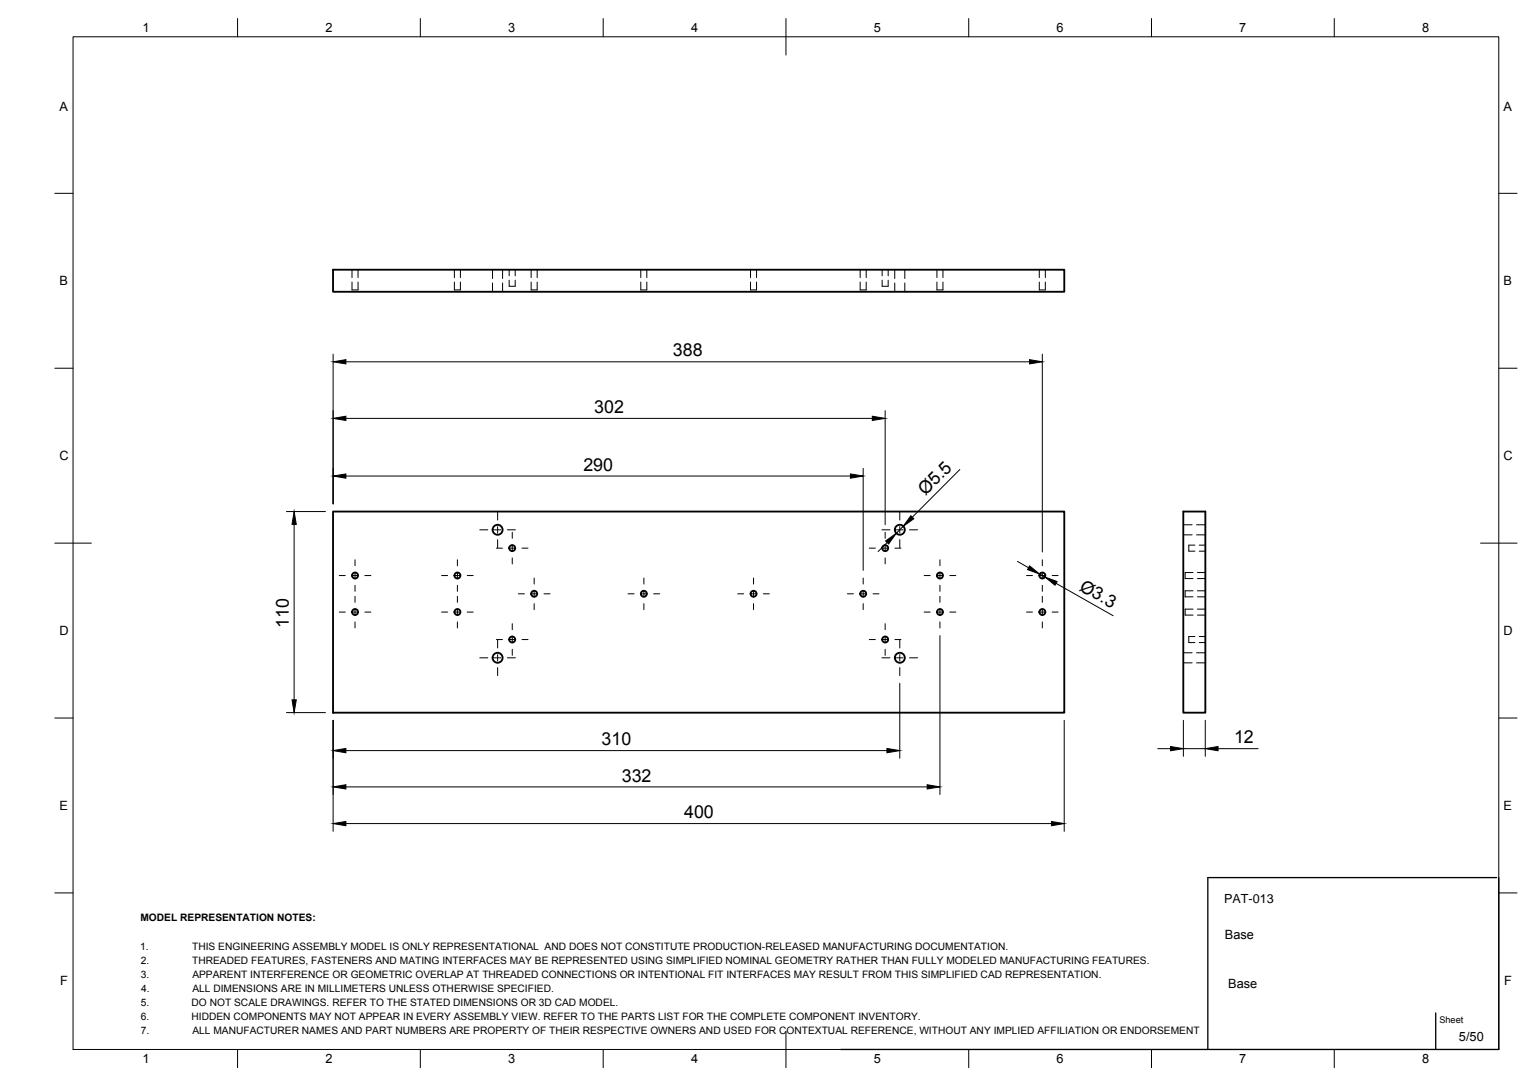
ISO-10303-21;
HEADER;
/* Generated by software containing ST-Developer
 * from STEP Tools, Inc. (www.steptools.com) 
 */

FILE_DESCRIPTION(
/* description */ ('Belt-driven linear axis on 2020 extrusion'),
/* implementation_level */ '2;1');

FILE_NAME(
/* name */ 'Base.step',
/* time_stamp */ '2026-10-28T03:26:09-07:00',
/* author */ (''),
/* organization */ (''),
/* preprocessor_version */ 'ST-DEVELOPER v20.2',
/* originating_system */ 'Autodesk Translation Framework v15.17.0.0',
/* authorisation */ '');

FILE_SCHEMA (('AUTOMOTIVE_DESIGN { 1 0 10303 214 3 1 1 }'));
ENDSEC;

DATA;
#10=MECHANICAL_DESIGN_GEOMETRIC_PRESENTATION_REPRESENTATION('',(#610),#20096);
#518=SHAPE_REPRESENTATION_RELATIONSHIP('SRR','None',#20314,#564);
#564=ADVANCED_BREP_SHAPE_REPRESENTATION('',(#666),#20045);
#610=STYLED_ITEM('',(#20629),#666);
#666=MANIFOLD_SOLID_BREP('Body1',#10923);
#718=FACE_BOUND('',#1913,.T.);
#719=FACE_BOUND('',#1914,.T.);
#720=FACE_BOUND('',#1915,.T.);
#721=FACE_BOUND('',#1916,.T.);
#722=FACE_BOUND('',#1917,.T.);
#723=FACE_BOUND('',#1918,.T.);
#724=FACE_BOUND('',#1919,.T.);
#725=FACE_BOUND('',#1920,.T.);
#726=FACE_BOUND('',#1921,.T.);
#727=FACE_BOUND('',#1922,.T.);
#728=FACE_BOUND('',#1923,.T.);
#729=FACE_BOUND('',#1924,.T.);
#730=FACE_BOUND('',#1925,.T.);
#731=FACE_BOUND('',#1926,.T.);
#732=FACE_BOUND('',#1927,.T.);
#733=FACE_BOUND('',#1928,.T.);
#734=FACE_BOUND('',#1929,.T.);
#735=FACE_BOUND('',#1930,.T.);
#736=FACE_BOUND('',#1931,.T.);
#737=FACE_BOUND('',#1932,.T.);
#738=FACE_BOUND('',#1934,.T.);
#739=FACE_BOUND('',#1935,.T.);
#740=FACE_BOUND('',#1936,.T.);
#741=FACE_BOUND('',#1937,.T.);
#889=PLANE('',#11496);
#890=PLANE('',#11500);
#891=PLANE('',#11504);
#892=PLANE('',#11508);
#893=PLANE('',#11512);
#894=PLANE('',#11516);
#895=PLANE('',#11520);
#896=PLANE('',#11524);
#897=PLANE('',#11540);
#898=PLANE('',#11544);
#899=PLANE('',#11548);
#900=PLANE('',#11552);
#901=PLANE('',#11556);
#902=PLANE('',#11560);
#903=PLANE('',#11564);
#904=PLANE('',#11568);
#905=PLANE('',#11569);
#906=PLANE('',#11570);
#907=PLANE('',#11571);
#908=PLANE('',#11572);
#909=PLANE('',#11573);
#910=PLANE('',#11574);
#1250=FACE_OUTER_BOUND('',#1872,.T.);
#1251=FACE_OUTER_BOUND('',#1873,.T.);
#1252=FACE_OUTER_BOUND('',#1874,.T.);
#1253=FACE_OUTER_BOUND('',#1875,.T.);
#1254=FACE_OUTER_BOUND('',#1876,.T.);
#1255=FACE_OUTER_BOUND('',#1877,.T.);
#1256=FACE_OUTER_BOUND('',#1878,.T.);
#1257=FACE_OUTER_BOUND('',#1879,.T.);
#1258=FACE_OUTER_BOUND('',#1880,.T.);
#1259=FACE_OUTER_BOUND('',#1881,.T.);
#1260=FACE_OUTER_BOUND('',#1882,.T.);
#1261=FACE_OUTER_BOUND('',#1883,.T.);
#1262=FACE_OUTER_BOUND('',#1884,.T.);
#1263=FACE_OUTER_BOUND('',#1885,.T.);
#1264=FACE_OUTER_BOUND('',#1886,.T.);
#1265=FACE_OUTER_BOUND('',#1887,.T.);
#1266=FACE_OUTER_BOUND('',#1888,.T.);
#1267=FACE_OUTER_BOUND('',#1889,.T.);
#1268=FACE_OUTER_BOUND('',#1890,.T.);
#1269=FACE_OUTER_BOUND('',#1891,.T.);
#1270=FACE_OUTER_BOUND('',#1892,.T.);
#1271=FACE_OUTER_BOUND('',#1893,.T.);
#1272=FACE_OUTER_BOUND('',#1894,.T.);
#1273=FACE_OUTER_BOUND('',#1895,.T.);
#1274=FACE_OUTER_BOUND('',#1896,.T.);
#1275=FACE_OUTER_BOUND('',#1897,.T.);
#1276=FACE_OUTER_BOUND('',#1898,.T.);
#1277=FACE_OUTER_BOUND('',#1899,.T.);
#1278=FACE_OUTER_BOUND('',#1900,.T.);
#1279=FACE_OUTER_BOUND('',#1901,.T.);
#1280=FACE_OUTER_BOUND('',#1902,.T.);
#1281=FACE_OUTER_BOUND('',#1903,.T.);
#1282=FACE_OUTER_BOUND('',#1904,.T.);
#1283=FACE_OUTER_BOUND('',#1905,.T.);
#1284=FACE_OUTER_BOUND('',#1906,.T.);
#1285=FACE_OUTER_BOUND('',#1907,.T.);
#1286=FACE_OUTER_BOUND('',#1908,.T.);
#1287=FACE_OUTER_BOUND('',#1909,.T.);
#1288=FACE_OUTER_BOUND('',#1910,.T.);
#1289=FACE_OUTER_BOUND('',#1911,.T.);
#1290=FACE_OUTER_BOUND('',#1912,.T.);
#1291=FACE_OUTER_BOUND('',#1933,.T.);
#1872=EDGE_LOOP('',(#7253,#7254,#7255,#7256));
#1873=EDGE_LOOP('',(#7257));
#1874=EDGE_LOOP('',(#7258,#7259,#7260,#7261));
#1875=EDGE_LOOP('',(#7262));
#1876=EDGE_LOOP('',(#7263,#7264,#7265,#7266));
#1877=EDGE_LOOP('',(#7267));
#1878=EDGE_LOOP('',(#7268,#7269,#7270,#7271));
#1879=EDGE_LOOP('',(#7272));
#1880=EDGE_LOOP('',(#7273,#7274,#7275,#7276));
#1881=EDGE_LOOP('',(#7277));
#1882=EDGE_LOOP('',(#7278,#7279,#7280,#7281));
#1883=EDGE_LOOP('',(#7282));
#1884=EDGE_LOOP('',(#7283,#7284,#7285,#7286));
#1885=EDGE_LOOP('',(#7287));
#1886=EDGE_LOOP('',(#7288,#7289,#7290,#7291));
#1887=EDGE_LOOP('',(#7292));
#1888=EDGE_LOOP('',(#7293,#7294,#7295,#7296));
#1889=EDGE_LOOP('',(#7297,#7298,#7299,#7300));
#1890=EDGE_LOOP('',(#7301,#7302,#7303,#7304));
#1891=EDGE_LOOP('',(#7305,#7306,#7307,#7308));
#1892=EDGE_LOOP('',(#7309,#7310,#7311,#7312));
#1893=EDGE_LOOP('',(#7313));
#1894=EDGE_LOOP('',(#7314,#7315,#7316,#7317));
#1895=EDGE_LOOP('',(#7318));
#1896=EDGE_LOOP('',(#7319,#7320,#7321,#7322));
#1897=EDGE_LOOP('',(#7323));
#1898=EDGE_LOOP('',(#7324,#7325,#7326,#7327));
#1899=EDGE_LOOP('',(#7328));
#1900=EDGE_LOOP('',(#7329,#7330,#7331,#7332));
#1901=EDGE_LOOP('',(#7333));
#1902=EDGE_LOOP('',(#7334,#7335,#7336,#7337));
#1903=EDGE_LOOP('',(#7338));
#1904=EDGE_LOOP('',(#7339,#7340,#7341,#7342));
#1905=EDGE_LOOP('',(#7343));
#1906=EDGE_LOOP('',(#7344,#7345,#7346,#7347));
#1907=EDGE_LOOP('',(#7348));
#1908=EDGE_LOOP('',(#7349,#7350,#7351,#7352));
#1909=EDGE_LOOP('',(#7353,#7354,#7355,#7356));
#1910=EDGE_LOOP('',(#7357,#7358,#7359,#7360));
#1911=EDGE_LOOP('',(#7361,#7362,#7363,#7364));
#1912=EDGE_LOOP('',(#7365,#7366,#7367,#7368));
#1913=EDGE_LOOP('',(#7369));
#1914=EDGE_LOOP('',(#7370));
#1915=EDGE_LOOP('',(#7371));
#1916=EDGE_LOOP('',(#7372));
#1917=EDGE_LOOP('',(#7373));
#1918=EDGE_LOOP('',(#7374));
#1919=EDGE_LOOP('',(#7375));
#1920=EDGE_LOOP('',(#7376));
#1921=EDGE_LOOP('',(#7377));
#1922=EDGE_LOOP('',(#7378));
#1923=EDGE_LOOP('',(#7379));
#1924=EDGE_LOOP('',(#7380));
#1925=EDGE_LOOP('',(#7381));
#1926=EDGE_LOOP('',(#7382));
#1927=EDGE_LOOP('',(#7383));
#1928=EDGE_LOOP('',(#7384));
#1929=EDGE_LOOP('',(#7385));
#1930=EDGE_LOOP('',(#7386));
#1931=EDGE_LOOP('',(#7387));
#1932=EDGE_LOOP('',(#7388));
#1933=EDGE_LOOP('',(#7389,#7390,#7391,#7392));
#1934=EDGE_LOOP('',(#7393));
#1935=EDGE_LOOP('',(#7394));
#1936=EDGE_LOOP('',(#7395));
#1937=EDGE_LOOP('',(#7396));
#2665=LINE('',#16239,#3522);
#2666=LINE('',#16246,#3523);
#2667=LINE('',#16253,#3524);
#2668=LINE('',#16260,#3525);
#2669=LINE('',#16267,#3526);
#2670=LINE('',#16274,#3527);
#2671=LINE('',#16281,#3528);
#2672=LINE('',#16288,#3529);
#2673=LINE('',#16295,#3530);
#2674=LINE('',#16301,#3531);
#2675=LINE('',#16307,#3532);
#2676=LINE('',#16313,#3533);
#2677=LINE('',#16319,#3534);
#2678=LINE('',#16326,#3535);
#2679=LINE('',#16333,#3536);
#2680=LINE('',#16340,#3537);
#2681=LINE('',#16347,#3538);
#2682=LINE('',#16354,#3539);
#2683=LINE('',#16361,#3540);
#2684=LINE('',#16368,#3541);
#2685=LINE('',#16374,#3542);
#2686=LINE('',#16376,#3543);
#2687=LINE('',#16378,#3544);
#2688=LINE('',#16379,#3545);
#2689=LINE('',#16382,#3546);
#2690=LINE('',#16384,#3547);
#2691=LINE('',#16385,#3548);
#2692=LINE('',#16388,#3549);
#2693=LINE('',#16390,#3550);
#2694=LINE('',#16391,#3551);
#2695=LINE('',#16393,#3552);
#2696=LINE('',#16394,#3553);
#3522=VECTOR('',#12795,0.164999999999999);
#3523=VECTOR('',#12804,0.164999999999999);
#3524=VECTOR('',#12813,0.165);
#3525=VECTOR('',#12822,0.165);
#3526=VECTOR('',#12831,0.164999999999999);
#3527=VECTOR('',#12840,0.164999999999999);
#3528=VECTOR('',#12849,0.164999999999999);
#3529=VECTOR('',#12858,0.165);
#3530=VECTOR('',#12867,0.274999999999999);
#3531=VECTOR('',#12874,0.275);
#3532=VECTOR('',#12881,0.274999999999999);
#3533=VECTOR('',#12888,0.275);
#3534=VECTOR('',#12895,0.164999999999999);
#3535=VECTOR('',#12904,0.164999999999999);
#3536=VECTOR('',#12913,0.164999999999999);
#3537=VECTOR('',#12922,0.164999999999999);
#3538=VECTOR('',#12931,0.165);
#3539=VECTOR('',#12940,0.165);
#3540=VECTOR('',#12949,0.165);
#3541=VECTOR('',#12958,0.165);
#3542=VECTOR('',#12965,1.);
#3543=VECTOR('',#12966,1.);
#3544=VECTOR('',#12967,1.);
#3545=VECTOR('',#12968,1.);
#3546=VECTOR('',#12971,1.);
#3547=VECTOR('',#12972,1.);
#3548=VECTOR('',#12973,1.);
#3549=VECTOR('',#12976,1.);
#3550=VECTOR('',#12977,1.);
#3551=VECTOR('',#12978,1.);
#3552=VECTOR('',#12981,1.);
#3553=VECTOR('',#12982,1.);
#4379=CIRCLE('',#11494,0.164999999999999);
#4380=CIRCLE('',#11495,0.164999999999999);
#4381=CIRCLE('',#11498,0.164999999999999);
#4382=CIRCLE('',#11499,0.164999999999999);
#4383=CIRCLE('',#11502,0.165);
#4384=CIRCLE('',#11503,0.165);
#4385=CIRCLE('',#11506,0.165);
#4386=CIRCLE('',#11507,0.165);
#4387=CIRCLE('',#11510,0.164999999999999);
#4388=CIRCLE('',#11511,0.164999999999999);
#4389=CIRCLE('',#11514,0.164999999999999);
#4390=CIRCLE('',#11515,0.164999999999999);
#4391=CIRCLE('',#11518,0.164999999999999);
#4392=CIRCLE('',#11519,0.164999999999999);
#4393=CIRCLE('',#11522,0.165);
#4394=CIRCLE('',#11523,0.165);
#4395=CIRCLE('',#11526,0.274999999999999);
#4396=CIRCLE('',#11527,0.274999999999999);
#4397=CIRCLE('',#11529,0.275);
#4398=CIRCLE('',#11530,0.275);
#4399=CIRCLE('',#11532,0.274999999999999);
#4400=CIRCLE('',#11533,0.274999999999999);
#4401=CIRCLE('',#11535,0.275);
#4402=CIRCLE('',#11536,0.275);
#4403=CIRCLE('',#11538,0.164999999999999);
#4404=CIRCLE('',#11539,0.164999999999999);
#4405=CIRCLE('',#11542,0.164999999999999);
#4406=CIRCLE('',#11543,0.164999999999999);
#4407=CIRCLE('',#11546,0.164999999999999);
#4408=CIRCLE('',#11547,0.164999999999999);
#4409=CIRCLE('',#11550,0.164999999999999);
#4410=CIRCLE('',#11551,0.164999999999999);
#4411=CIRCLE('',#11554,0.165);
#4412=CIRCLE('',#11555,0.165);
#4413=CIRCLE('',#11558,0.165);
#4414=CIRCLE('',#11559,0.165);
#4415=CIRCLE('',#11562,0.165);
#4416=CIRCLE('',#11563,0.165);
#4417=CIRCLE('',#11566,0.165);
#4418=CIRCLE('',#11567,0.165);
#4892=VERTEX_POINT('',#16236);
#4893=VERTEX_POINT('',#16238);
#4894=VERTEX_POINT('',#16243);
#4895=VERTEX_POINT('',#16245);
#4896=VERTEX_POINT('',#16250);
#4897=VERTEX_POINT('',#16252);
#4898=VERTEX_POINT('',#16257);
#4899=VERTEX_POINT('',#16259);
#4900=VERTEX_POINT('',#16264);
#4901=VERTEX_POINT('',#16266);
#4902=VERTEX_POINT('',#16271);
#4903=VERTEX_POINT('',#16273);
#4904=VERTEX_POINT('',#16278);
#4905=VERTEX_POINT('',#16280);
#4906=VERTEX_POINT('',#16285);
#4907=VERTEX_POINT('',#16287);
#4908=VERTEX_POINT('',#16292);
#4909=VERTEX_POINT('',#16294);
#4910=VERTEX_POINT('',#16298);
#4911=VERTEX_POINT('',#16300);
#4912=VERTEX_POINT('',#16304);
#4913=VERTEX_POINT('',#16306);
#4914=VERTEX_POINT('',#16310);
#4915=VERTEX_POINT('',#16312);
#4916=VERTEX_POINT('',#16316);
#4917=VERTEX_POINT('',#16318);
#4918=VERTEX_POINT('',#16323);
#4919=VERTEX_POINT('',#16325);
#4920=VERTEX_POINT('',#16330);
#4921=VERTEX_POINT('',#16332);
#4922=VERTEX_POINT('',#16337);
#4923=VERTEX_POINT('',#16339);
#4924=VERTEX_POINT('',#16344);
#4925=VERTEX_POINT('',#16346);
#4926=VERTEX_POINT('',#16351);
#4927=VERTEX_POINT('',#16353);
#4928=VERTEX_POINT('',#16358);
#4929=VERTEX_POINT('',#16360);
#4930=VERTEX_POINT('',#16365);
#4931=VERTEX_POINT('',#16367);
#4932=VERTEX_POINT('',#16372);
#4933=VERTEX_POINT('',#16373);
#4934=VERTEX_POINT('',#16375);
#4935=VERTEX_POINT('',#16377);
#4936=VERTEX_POINT('',#16381);
#4937=VERTEX_POINT('',#16383);
#4938=VERTEX_POINT('',#16387);
#4939=VERTEX_POINT('',#16389);
#5841=EDGE_CURVE('',#4892,#4892,#4379,.T.);
#5842=EDGE_CURVE('',#4892,#4893,#2665,.T.);
#5843=EDGE_CURVE('',#4893,#4893,#4380,.T.);
#5844=EDGE_CURVE('',#4894,#4894,#4381,.T.);
#5845=EDGE_CURVE('',#4894,#4895,#2666,.T.);
#5846=EDGE_CURVE('',#4895,#4895,#4382,.T.);
#5847=EDGE_CURVE('',#4896,#4896,#4383,.T.);
#5848=EDGE_CURVE('',#4896,#4897,#2667,.T.);
#5849=EDGE_CURVE('',#4897,#4897,#4384,.T.);
#5850=EDGE_CURVE('',#4898,#4898,#4385,.T.);
#5851=EDGE_CURVE('',#4898,#4899,#2668,.T.);
#5852=EDGE_CURVE('',#4899,#4899,#4386,.T.);
#5853=EDGE_CURVE('',#4900,#4900,#4387,.T.);
#5854=EDGE_CURVE('',#4900,#4901,#2669,.T.);
#5855=EDGE_CURVE('',#4901,#4901,#4388,.T.);
#5856=EDGE_CURVE('',#4902,#4902,#4389,.T.);
#5857=EDGE_CURVE('',#4902,#4903,#2670,.T.);
#5858=EDGE_CURVE('',#4903,#4903,#4390,.T.);
#5859=EDGE_CURVE('',#4904,#4904,#4391,.T.);
#5860=EDGE_CURVE('',#4904,#4905,#2671,.T.);
#5861=EDGE_CURVE('',#4905,#4905,#4392,.T.);
#5862=EDGE_CURVE('',#4906,#4906,#4393,.T.);
#5863=EDGE_CURVE('',#4906,#4907,#2672,.T.);
#5864=EDGE_CURVE('',#4907,#4907,#4394,.T.);
#5865=EDGE_CURVE('',#4908,#4908,#4395,.T.);
#5866=EDGE_CURVE('',#4908,#4909,#2673,.T.);
#5867=EDGE_CURVE('',#4909,#4909,#4396,.T.);
#5868=EDGE_CURVE('',#4910,#4910,#4397,.T.);
#5869=EDGE_CURVE('',#4910,#4911,#2674,.T.);
#5870=EDGE_CURVE('',#4911,#4911,#4398,.T.);
#5871=EDGE_CURVE('',#4912,#4912,#4399,.T.);
#5872=EDGE_CURVE('',#4912,#4913,#2675,.T.);
#5873=EDGE_CURVE('',#4913,#4913,#4400,.T.);
#5874=EDGE_CURVE('',#4914,#4914,#4401,.T.);
#5875=EDGE_CURVE('',#4914,#4915,#2676,.T.);
#5876=EDGE_CURVE('',#4915,#4915,#4402,.T.);
#5877=EDGE_CURVE('',#4916,#4916,#4403,.T.);
#5878=EDGE_CURVE('',#4916,#4917,#2677,.T.);
#5879=EDGE_CURVE('',#4917,#4917,#4404,.T.);
#5880=EDGE_CURVE('',#4918,#4918,#4405,.T.);
#5881=EDGE_CURVE('',#4918,#4919,#2678,.T.);
#5882=EDGE_CURVE('',#4919,#4919,#4406,.T.);
#5883=EDGE_CURVE('',#4920,#4920,#4407,.T.);
#5884=EDGE_CURVE('',#4920,#4921,#2679,.T.);
#5885=EDGE_CURVE('',#4921,#4921,#4408,.T.);
#5886=EDGE_CURVE('',#4922,#4922,#4409,.T.);
#5887=EDGE_CURVE('',#4922,#4923,#2680,.T.);
#5888=EDGE_CURVE('',#4923,#4923,#4410,.T.);
#5889=EDGE_CURVE('',#4924,#4924,#4411,.T.);
#5890=EDGE_CURVE('',#4924,#4925,#2681,.T.);
#5891=EDGE_CURVE('',#4925,#4925,#4412,.T.);
#5892=EDGE_CURVE('',#4926,#4926,#4413,.T.);
#5893=EDGE_CURVE('',#4926,#4927,#2682,.T.);
#5894=EDGE_CURVE('',#4927,#4927,#4414,.T.);
#5895=EDGE_CURVE('',#4928,#4928,#4415,.T.);
#5896=EDGE_CURVE('',#4928,#4929,#2683,.T.);
#5897=EDGE_CURVE('',#4929,#4929,#4416,.T.);
#5898=EDGE_CURVE('',#4930,#4930,#4417,.T.);
#5899=EDGE_CURVE('',#4930,#4931,#2684,.T.);
#5900=EDGE_CURVE('',#4931,#4931,#4418,.T.);
#5901=EDGE_CURVE('',#4932,#4933,#2685,.T.);
#5902=EDGE_CURVE('',#4933,#4934,#2686,.T.);
#5903=EDGE_CURVE('',#4935,#4934,#2687,.T.);
#5904=EDGE_CURVE('',#4932,#4935,#2688,.T.);
#5905=EDGE_CURVE('',#4936,#4932,#2689,.T.);
#5906=EDGE_CURVE('',#4937,#4935,#2690,.T.);
#5907=EDGE_CURVE('',#4936,#4937,#2691,.T.);
#5908=EDGE_CURVE('',#4938,#4936,#2692,.T.);
#5909=EDGE_CURVE('',#4939,#4937,#2693,.T.);
#5910=EDGE_CURVE('',#4938,#4939,#2694,.T.);
#5911=EDGE_CURVE('',#4933,#4938,#2695,.T.);
#5912=EDGE_CURVE('',#4934,#4939,#2696,.T.);
#7253=ORIENTED_EDGE('',*,*,#5841,.F.);
#7254=ORIENTED_EDGE('',*,*,#5842,.T.);
#7255=ORIENTED_EDGE('',*,*,#5843,.F.);
#7256=ORIENTED_EDGE('',*,*,#5842,.F.);
#7257=ORIENTED_EDGE('',*,*,#5841,.T.);
#7258=ORIENTED_EDGE('',*,*,#5844,.F.);
#7259=ORIENTED_EDGE('',*,*,#5845,.T.);
#7260=ORIENTED_EDGE('',*,*,#5846,.F.);
#7261=ORIENTED_EDGE('',*,*,#5845,.F.);
#7262=ORIENTED_EDGE('',*,*,#5844,.T.);
#7263=ORIENTED_EDGE('',*,*,#5847,.F.);
#7264=ORIENTED_EDGE('',*,*,#5848,.T.);
#7265=ORIENTED_EDGE('',*,*,#5849,.F.);
#7266=ORIENTED_EDGE('',*,*,#5848,.F.);
#7267=ORIENTED_EDGE('',*,*,#5847,.T.);
#7268=ORIENTED_EDGE('',*,*,#5850,.F.);
#7269=ORIENTED_EDGE('',*,*,#5851,.T.);
#7270=ORIENTED_EDGE('',*,*,#5852,.F.);
#7271=ORIENTED_EDGE('',*,*,#5851,.F.);
#7272=ORIENTED_EDGE('',*,*,#5850,.T.);
#7273=ORIENTED_EDGE('',*,*,#5853,.F.);
#7274=ORIENTED_EDGE('',*,*,#5854,.T.);
#7275=ORIENTED_EDGE('',*,*,#5855,.F.);
#7276=ORIENTED_EDGE('',*,*,#5854,.F.);
#7277=ORIENTED_EDGE('',*,*,#5853,.T.);
#7278=ORIENTED_EDGE('',*,*,#5856,.F.);
#7279=ORIENTED_EDGE('',*,*,#5857,.T.);
#7280=ORIENTED_EDGE('',*,*,#5858,.F.);
#7281=ORIENTED_EDGE('',*,*,#5857,.F.);
#7282=ORIENTED_EDGE('',*,*,#5856,.T.);
#7283=ORIENTED_EDGE('',*,*,#5859,.F.);
#7284=ORIENTED_EDGE('',*,*,#5860,.T.);
#7285=ORIENTED_EDGE('',*,*,#5861,.F.);
#7286=ORIENTED_EDGE('',*,*,#5860,.F.);
#7287=ORIENTED_EDGE('',*,*,#5859,.T.);
#7288=ORIENTED_EDGE('',*,*,#5862,.F.);
#7289=ORIENTED_EDGE('',*,*,#5863,.T.);
#7290=ORIENTED_EDGE('',*,*,#5864,.F.);
#7291=ORIENTED_EDGE('',*,*,#5863,.F.);
#7292=ORIENTED_EDGE('',*,*,#5862,.T.);
#7293=ORIENTED_EDGE('',*,*,#5865,.F.);
#7294=ORIENTED_EDGE('',*,*,#5866,.T.);
#7295=ORIENTED_EDGE('',*,*,#5867,.F.);
#7296=ORIENTED_EDGE('',*,*,#5866,.F.);
#7297=ORIENTED_EDGE('',*,*,#5868,.F.);
#7298=ORIENTED_EDGE('',*,*,#5869,.T.);
#7299=ORIENTED_EDGE('',*,*,#5870,.F.);
#7300=ORIENTED_EDGE('',*,*,#5869,.F.);
#7301=ORIENTED_EDGE('',*,*,#5871,.F.);
#7302=ORIENTED_EDGE('',*,*,#5872,.T.);
#7303=ORIENTED_EDGE('',*,*,#5873,.F.);
#7304=ORIENTED_EDGE('',*,*,#5872,.F.);
#7305=ORIENTED_EDGE('',*,*,#5874,.F.);
#7306=ORIENTED_EDGE('',*,*,#5875,.T.);
#7307=ORIENTED_EDGE('',*,*,#5876,.F.);
#7308=ORIENTED_EDGE('',*,*,#5875,.F.);
#7309=ORIENTED_EDGE('',*,*,#5877,.F.);
#7310=ORIENTED_EDGE('',*,*,#5878,.T.);
#7311=ORIENTED_EDGE('',*,*,#5879,.F.);
#7312=ORIENTED_EDGE('',*,*,#5878,.F.);
#7313=ORIENTED_EDGE('',*,*,#5877,.T.);
#7314=ORIENTED_EDGE('',*,*,#5880,.F.);
#7315=ORIENTED_EDGE('',*,*,#5881,.T.);
#7316=ORIENTED_EDGE('',*,*,#5882,.F.);
#7317=ORIENTED_EDGE('',*,*,#5881,.F.);
#7318=ORIENTED_EDGE('',*,*,#5880,.T.);
#7319=ORIENTED_EDGE('',*,*,#5883,.F.);
#7320=ORIENTED_EDGE('',*,*,#5884,.T.);
#7321=ORIENTED_EDGE('',*,*,#5885,.F.);
#7322=ORIENTED_EDGE('',*,*,#5884,.F.);
#7323=ORIENTED_EDGE('',*,*,#5883,.T.);
#7324=ORIENTED_EDGE('',*,*,#5886,.F.);
#7325=ORIENTED_EDGE('',*,*,#5887,.T.);
#7326=ORIENTED_EDGE('',*,*,#5888,.F.);
#7327=ORIENTED_EDGE('',*,*,#5887,.F.);
#7328=ORIENTED_EDGE('',*,*,#5886,.T.);
#7329=ORIENTED_EDGE('',*,*,#5889,.F.);
#7330=ORIENTED_EDGE('',*,*,#5890,.T.);
#7331=ORIENTED_EDGE('',*,*,#5891,.F.);
#7332=ORIENTED_EDGE('',*,*,#5890,.F.);
#7333=ORIENTED_EDGE('',*,*,#5889,.T.);
#7334=ORIENTED_EDGE('',*,*,#5892,.F.);
#7335=ORIENTED_EDGE('',*,*,#5893,.T.);
#7336=ORIENTED_EDGE('',*,*,#5894,.F.);
#7337=ORIENTED_EDGE('',*,*,#5893,.F.);
#7338=ORIENTED_EDGE('',*,*,#5892,.T.);
#7339=ORIENTED_EDGE('',*,*,#5895,.F.);
#7340=ORIENTED_EDGE('',*,*,#5896,.T.);
#7341=ORIENTED_EDGE('',*,*,#5897,.F.);
#7342=ORIENTED_EDGE('',*,*,#5896,.F.);
#7343=ORIENTED_EDGE('',*,*,#5895,.T.);
#7344=ORIENTED_EDGE('',*,*,#5898,.F.);
#7345=ORIENTED_EDGE('',*,*,#5899,.T.);
#7346=ORIENTED_EDGE('',*,*,#5900,.F.);
#7347=ORIENTED_EDGE('',*,*,#5899,.F.);
#7348=ORIENTED_EDGE('',*,*,#5898,.T.);
#7349=ORIENTED_EDGE('',*,*,#5901,.T.);
#7350=ORIENTED_EDGE('',*,*,#5902,.T.);
#7351=ORIENTED_EDGE('',*,*,#5903,.F.);
#7352=ORIENTED_EDGE('',*,*,#5904,.F.);
#7353=ORIENTED_EDGE('',*,*,#5905,.T.);
#7354=ORIENTED_EDGE('',*,*,#5904,.T.);
#7355=ORIENTED_EDGE('',*,*,#5906,.F.);
#7356=ORIENTED_EDGE('',*,*,#5907,.F.);
#7357=ORIENTED_EDGE('',*,*,#5908,.T.);
#7358=ORIENTED_EDGE('',*,*,#5907,.T.);
#7359=ORIENTED_EDGE('',*,*,#5909,.F.);
#7360=ORIENTED_EDGE('',*,*,#5910,.F.);
#7361=ORIENTED_EDGE('',*,*,#5911,.T.);
#7362=ORIENTED_EDGE('',*,*,#5910,.T.);
#7363=ORIENTED_EDGE('',*,*,#5912,.F.);
#7364=ORIENTED_EDGE('',*,*,#5902,.F.);
#7365=ORIENTED_EDGE('',*,*,#5912,.T.);
#7366=ORIENTED_EDGE('',*,*,#5909,.T.);
#7367=ORIENTED_EDGE('',*,*,#5906,.T.);
#7368=ORIENTED_EDGE('',*,*,#5903,.T.);
#7369=ORIENTED_EDGE('',*,*,#5849,.T.);
#7370=ORIENTED_EDGE('',*,*,#5852,.T.);
#7371=ORIENTED_EDGE('',*,*,#5858,.T.);
#7372=ORIENTED_EDGE('',*,*,#5864,.T.);
#7373=ORIENTED_EDGE('',*,*,#5870,.T.);
#7374=ORIENTED_EDGE('',*,*,#5876,.T.);
#7375=ORIENTED_EDGE('',*,*,#5900,.T.);
#7376=ORIENTED_EDGE('',*,*,#5897,.T.);
#7377=ORIENTED_EDGE('',*,*,#5894,.T.);
#7378=ORIENTED_EDGE('',*,*,#5891,.T.);
#7379=ORIENTED_EDGE('',*,*,#5888,.T.);
#7380=ORIENTED_EDGE('',*,*,#5885,.T.);
#7381=ORIENTED_EDGE('',*,*,#5882,.T.);
#7382=ORIENTED_EDGE('',*,*,#5879,.T.);
#7383=ORIENTED_EDGE('',*,*,#5873,.T.);
#7384=ORIENTED_EDGE('',*,*,#5867,.T.);
#7385=ORIENTED_EDGE('',*,*,#5861,.T.);
#7386=ORIENTED_EDGE('',*,*,#5855,.T.);
#7387=ORIENTED_EDGE('',*,*,#5846,.T.);
#7388=ORIENTED_EDGE('',*,*,#5843,.T.);
#7389=ORIENTED_EDGE('',*,*,#5911,.F.);
#7390=ORIENTED_EDGE('',*,*,#5901,.F.);
#7391=ORIENTED_EDGE('',*,*,#5905,.F.);
#7392=ORIENTED_EDGE('',*,*,#5908,.F.);
#7393=ORIENTED_EDGE('',*,*,#5865,.T.);
#7394=ORIENTED_EDGE('',*,*,#5868,.T.);
#7395=ORIENTED_EDGE('',*,*,#5871,.T.);
#7396=ORIENTED_EDGE('',*,*,#5874,.T.);
#10077=CYLINDRICAL_SURFACE('',#11493,0.164999999999999);
#10078=CYLINDRICAL_SURFACE('',#11497,0.164999999999999);
#10079=CYLINDRICAL_SURFACE('',#11501,0.165);
#10080=CYLINDRICAL_SURFACE('',#11505,0.165);
#10081=CYLINDRICAL_SURFACE('',#11509,0.164999999999999);
#10082=CYLINDRICAL_SURFACE('',#11513,0.164999999999999);
#10083=CYLINDRICAL_SURFACE('',#11517,0.164999999999999);
#10084=CYLINDRICAL_SURFACE('',#11521,0.165);
#10085=CYLINDRICAL_SURFACE('',#11525,0.274999999999999);
#10086=CYLINDRICAL_SURFACE('',#11528,0.275);
#10087=CYLINDRICAL_SURFACE('',#11531,0.274999999999999);
#10088=CYLINDRICAL_SURFACE('',#11534,0.275);
#10089=CYLINDRICAL_SURFACE('',#11537,0.164999999999999);
#10090=CYLINDRICAL_SURFACE('',#11541,0.164999999999999);
#10091=CYLINDRICAL_SURFACE('',#11545,0.164999999999999);
#10092=CYLINDRICAL_SURFACE('',#11549,0.164999999999999);
#10093=CYLINDRICAL_SURFACE('',#11553,0.165);
#10094=CYLINDRICAL_SURFACE('',#11557,0.165);
#10095=CYLINDRICAL_SURFACE('',#11561,0.165);
#10096=CYLINDRICAL_SURFACE('',#11565,0.165);
#10301=ADVANCED_FACE('',(#1250),#10077,.F.);
#10302=ADVANCED_FACE('',(#1251),#889,.T.);
#10303=ADVANCED_FACE('',(#1252),#10078,.F.);
#10304=ADVANCED_FACE('',(#1253),#890,.T.);
#10305=ADVANCED_FACE('',(#1254),#10079,.F.);
#10306=ADVANCED_FACE('',(#1255),#891,.T.);
#10307=ADVANCED_FACE('',(#1256),#10080,.F.);
#10308=ADVANCED_FACE('',(#1257),#892,.T.);
#10309=ADVANCED_FACE('',(#1258),#10081,.F.);
#10310=ADVANCED_FACE('',(#1259),#893,.T.);
#10311=ADVANCED_FACE('',(#1260),#10082,.F.);
#10312=ADVANCED_FACE('',(#1261),#894,.T.);
#10313=ADVANCED_FACE('',(#1262),#10083,.F.);
#10314=ADVANCED_FACE('',(#1263),#895,.T.);
#10315=ADVANCED_FACE('',(#1264),#10084,.F.);
#10316=ADVANCED_FACE('',(#1265),#896,.T.);
#10317=ADVANCED_FACE('',(#1266),#10085,.F.);
#10318=ADVANCED_FACE('',(#1267),#10086,.F.);
#10319=ADVANCED_FACE('',(#1268),#10087,.F.);
#10320=ADVANCED_FACE('',(#1269),#10088,.F.);
#10321=ADVANCED_FACE('',(#1270),#10089,.F.);
#10322=ADVANCED_FACE('',(#1271),#897,.T.);
#10323=ADVANCED_FACE('',(#1272),#10090,.F.);
#10324=ADVANCED_FACE('',(#1273),#898,.T.);
#10325=ADVANCED_FACE('',(#1274),#10091,.F.);
#10326=ADVANCED_FACE('',(#1275),#899,.T.);
#10327=ADVANCED_FACE('',(#1276),#10092,.F.);
#10328=ADVANCED_FACE('',(#1277),#900,.T.);
#10329=ADVANCED_FACE('',(#1278),#10093,.F.);
#10330=ADVANCED_FACE('',(#1279),#901,.T.);
#10331=ADVANCED_FACE('',(#1280),#10094,.F.);
#10332=ADVANCED_FACE('',(#1281),#902,.T.);
#10333=ADVANCED_FACE('',(#1282),#10095,.F.);
#10334=ADVANCED_FACE('',(#1283),#903,.T.);
#10335=ADVANCED_FACE('',(#1284),#10096,.F.);
#10336=ADVANCED_FACE('',(#1285),#904,.T.);
#10337=ADVANCED_FACE('',(#1286),#905,.T.);
#10338=ADVANCED_FACE('',(#1287),#906,.T.);
#10339=ADVANCED_FACE('',(#1288),#907,.T.);
#10340=ADVANCED_FACE('',(#1289),#908,.T.);
#10341=ADVANCED_FACE('',(#1290,#718,#719,#720,#721,#722,#723,#724,#725,
#726,#727,#728,#729,#730,#731,#732,#733,#734,#735,#736,#737),#909,.T.);
#10342=ADVANCED_FACE('',(#1291,#738,#739,#740,#741),#910,.F.);
#10923=CLOSED_SHELL('',(#10301,#10302,#10303,#10304,#10305,#10306,#10307,
#10308,#10309,#10310,#10311,#10312,#10313,#10314,#10315,#10316,#10317,#10318,
#10319,#10320,#10321,#10322,#10323,#10324,#10325,#10326,#10327,#10328,#10329,
#10330,#10331,#10332,#10333,#10334,#10335,#10336,#10337,#10338,#10339,#10340,
#10341,#10342));
#11492=AXIS2_PLACEMENT_3D('',#16234,#12789,#12790);
#11493=AXIS2_PLACEMENT_3D('',#16235,#12791,#12792);
#11494=AXIS2_PLACEMENT_3D('',#16237,#12793,#12794);
#11495=AXIS2_PLACEMENT_3D('',#16240,#12796,#12797);
#11496=AXIS2_PLACEMENT_3D('',#16241,#12798,#12799);
#11497=AXIS2_PLACEMENT_3D('',#16242,#12800,#12801);
#11498=AXIS2_PLACEMENT_3D('',#16244,#12802,#12803);
#11499=AXIS2_PLACEMENT_3D('',#16247,#12805,#12806);
#11500=AXIS2_PLACEMENT_3D('',#16248,#12807,#12808);
#11501=AXIS2_PLACEMENT_3D('',#16249,#12809,#12810);
#11502=AXIS2_PLACEMENT_3D('',#16251,#12811,#12812);
#11503=AXIS2_PLACEMENT_3D('',#16254,#12814,#12815);
#11504=AXIS2_PLACEMENT_3D('',#16255,#12816,#12817);
#11505=AXIS2_PLACEMENT_3D('',#16256,#12818,#12819);
#11506=AXIS2_PLACEMENT_3D('',#16258,#12820,#12821);
#11507=AXIS2_PLACEMENT_3D('',#16261,#12823,#12824);
#11508=AXIS2_PLACEMENT_3D('',#16262,#12825,#12826);
#11509=AXIS2_PLACEMENT_3D('',#16263,#12827,#12828);
#11510=AXIS2_PLACEMENT_3D('',#16265,#12829,#12830);
#11511=AXIS2_PLACEMENT_3D('',#16268,#12832,#12833);
#11512=AXIS2_PLACEMENT_3D('',#16269,#12834,#12835);
#11513=AXIS2_PLACEMENT_3D('',#16270,#12836,#12837);
#11514=AXIS2_PLACEMENT_3D('',#16272,#12838,#12839);
#11515=AXIS2_PLACEMENT_3D('',#16275,#12841,#12842);
#11516=AXIS2_PLACEMENT_3D('',#16276,#12843,#12844);
#11517=AXIS2_PLACEMENT_3D('',#16277,#12845,#12846);
#11518=AXIS2_PLACEMENT_3D('',#16279,#12847,#12848);
#11519=AXIS2_PLACEMENT_3D('',#16282,#12850,#12851);
#11520=AXIS2_PLACEMENT_3D('',#16283,#12852,#12853);
#11521=AXIS2_PLACEMENT_3D('',#16284,#12854,#12855);
#11522=AXIS2_PLACEMENT_3D('',#16286,#12856,#12857);
#11523=AXIS2_PLACEMENT_3D('',#16289,#12859,#12860);
#11524=AXIS2_PLACEMENT_3D('',#16290,#12861,#12862);
#11525=AXIS2_PLACEMENT_3D('',#16291,#12863,#12864);
#11526=AXIS2_PLACEMENT_3D('',#16293,#12865,#12866);
#11527=AXIS2_PLACEMENT_3D('',#16296,#12868,#12869);
#11528=AXIS2_PLACEMENT_3D('',#16297,#12870,#12871);
#11529=AXIS2_PLACEMENT_3D('',#16299,#12872,#12873);
#11530=AXIS2_PLACEMENT_3D('',#16302,#12875,#12876);
#11531=AXIS2_PLACEMENT_3D('',#16303,#12877,#12878);
#11532=AXIS2_PLACEMENT_3D('',#16305,#12879,#12880);
#11533=AXIS2_PLACEMENT_3D('',#16308,#12882,#12883);
#11534=AXIS2_PLACEMENT_3D('',#16309,#12884,#12885);
#11535=AXIS2_PLACEMENT_3D('',#16311,#12886,#12887);
#11536=AXIS2_PLACEMENT_3D('',#16314,#12889,#12890);
#11537=AXIS2_PLACEMENT_3D('',#16315,#12891,#12892);
#11538=AXIS2_PLACEMENT_3D('',#16317,#12893,#12894);
#11539=AXIS2_PLACEMENT_3D('',#16320,#12896,#12897);
#11540=AXIS2_PLACEMENT_3D('',#16321,#12898,#12899);
#11541=AXIS2_PLACEMENT_3D('',#16322,#12900,#12901);
#11542=AXIS2_PLACEMENT_3D('',#16324,#12902,#12903);
#11543=AXIS2_PLACEMENT_3D('',#16327,#12905,#12906);
#11544=AXIS2_PLACEMENT_3D('',#16328,#12907,#12908);
#11545=AXIS2_PLACEMENT_3D('',#16329,#12909,#12910);
#11546=AXIS2_PLACEMENT_3D('',#16331,#12911,#12912);
#11547=AXIS2_PLACEMENT_3D('',#16334,#12914,#12915);
#11548=AXIS2_PLACEMENT_3D('',#16335,#12916,#12917);
#11549=AXIS2_PLACEMENT_3D('',#16336,#12918,#12919);
#11550=AXIS2_PLACEMENT_3D('',#16338,#12920,#12921);
#11551=AXIS2_PLACEMENT_3D('',#16341,#12923,#12924);
#11552=AXIS2_PLACEMENT_3D('',#16342,#12925,#12926);
#11553=AXIS2_PLACEMENT_3D('',#16343,#12927,#12928);
#11554=AXIS2_PLACEMENT_3D('',#16345,#12929,#12930);
#11555=AXIS2_PLACEMENT_3D('',#16348,#12932,#12933);
#11556=AXIS2_PLACEMENT_3D('',#16349,#12934,#12935);
#11557=AXIS2_PLACEMENT_3D('',#16350,#12936,#12937);
#11558=AXIS2_PLACEMENT_3D('',#16352,#12938,#12939);
#11559=AXIS2_PLACEMENT_3D('',#16355,#12941,#12942);
#11560=AXIS2_PLACEMENT_3D('',#16356,#12943,#12944);
#11561=AXIS2_PLACEMENT_3D('',#16357,#12945,#12946);
#11562=AXIS2_PLACEMENT_3D('',#16359,#12947,#12948);
#11563=AXIS2_PLACEMENT_3D('',#16362,#12950,#12951);
#11564=AXIS2_PLACEMENT_3D('',#16363,#12952,#12953);
#11565=AXIS2_PLACEMENT_3D('',#16364,#12954,#12955);
#11566=AXIS2_PLACEMENT_3D('',#16366,#12956,#12957);
#11567=AXIS2_PLACEMENT_3D('',#16369,#12959,#12960);
#11568=AXIS2_PLACEMENT_3D('',#16370,#12961,#12962);
#11569=AXIS2_PLACEMENT_3D('',#16371,#12963,#12964);
#11570=AXIS2_PLACEMENT_3D('',#16380,#12969,#12970);
#11571=AXIS2_PLACEMENT_3D('',#16386,#12974,#12975);
#11572=AXIS2_PLACEMENT_3D('',#16392,#12979,#12980);
#11573=AXIS2_PLACEMENT_3D('',#16395,#12983,#12984);
#11574=AXIS2_PLACEMENT_3D('',#16396,#12985,#12986);
#12789=DIRECTION('axis',(0.,0.,1.));
#12790=DIRECTION('refdir',(1.,0.,0.));
#12791=DIRECTION('center_axis',(0.,0.,1.));
#12792=DIRECTION('ref_axis',(1.,0.,0.));
#12793=DIRECTION('center_axis',(0.,0.,1.));
#12794=DIRECTION('ref_axis',(1.,0.,0.));
#12795=DIRECTION('',(0.,0.,1.));
#12796=DIRECTION('center_axis',(0.,0.,-1.));
#12797=DIRECTION('ref_axis',(1.,0.,0.));
#12798=DIRECTION('center_axis',(0.,0.,1.));
#12799=DIRECTION('ref_axis',(1.,0.,0.));
#12800=DIRECTION('center_axis',(0.,0.,1.));
#12801=DIRECTION('ref_axis',(1.,0.,0.));
#12802=DIRECTION('center_axis',(0.,0.,1.));
#12803=DIRECTION('ref_axis',(1.,0.,0.));
#12804=DIRECTION('',(0.,0.,1.));
#12805=DIRECTION('center_axis',(0.,0.,-1.));
#12806=DIRECTION('ref_axis',(1.,0.,0.));
#12807=DIRECTION('center_axis',(0.,0.,1.));
#12808=DIRECTION('ref_axis',(1.,0.,0.));
#12809=DIRECTION('center_axis',(0.,0.,1.));
#12810=DIRECTION('ref_axis',(1.,0.,0.));
#12811=DIRECTION('center_axis',(0.,0.,1.));
#12812=DIRECTION('ref_axis',(1.,0.,0.));
#12813=DIRECTION('',(0.,0.,1.));
#12814=DIRECTION('center_axis',(0.,0.,-1.));
#12815=DIRECTION('ref_axis',(1.,0.,0.));
#12816=DIRECTION('center_axis',(0.,0.,1.));
#12817=DIRECTION('ref_axis',(1.,0.,0.));
#12818=DIRECTION('center_axis',(0.,0.,1.));
#12819=DIRECTION('ref_axis',(1.,0.,0.));
#12820=DIRECTION('center_axis',(0.,0.,1.));
#12821=DIRECTION('ref_axis',(1.,0.,0.));
#12822=DIRECTION('',(0.,0.,1.));
#12823=DIRECTION('center_axis',(0.,0.,-1.));
#12824=DIRECTION('ref_axis',(1.,0.,0.));
#12825=DIRECTION('center_axis',(0.,0.,1.));
#12826=DIRECTION('ref_axis',(1.,0.,0.));
#12827=DIRECTION('center_axis',(0.,0.,1.));
#12828=DIRECTION('ref_axis',(1.,0.,0.));
#12829=DIRECTION('center_axis',(0.,0.,1.));
#12830=DIRECTION('ref_axis',(1.,0.,0.));
#12831=DIRECTION('',(0.,0.,1.));
#12832=DIRECTION('center_axis',(0.,0.,-1.));
#12833=DIRECTION('ref_axis',(1.,0.,0.));
#12834=DIRECTION('center_axis',(0.,0.,1.));
#12835=DIRECTION('ref_axis',(1.,0.,0.));
#12836=DIRECTION('center_axis',(0.,0.,1.));
#12837=DIRECTION('ref_axis',(1.,0.,0.));
#12838=DIRECTION('center_axis',(0.,0.,1.));
#12839=DIRECTION('ref_axis',(1.,0.,0.));
#12840=DIRECTION('',(0.,0.,1.));
#12841=DIRECTION('center_axis',(0.,0.,-1.));
#12842=DIRECTION('ref_axis',(1.,0.,0.));
#12843=DIRECTION('center_axis',(0.,0.,1.));
#12844=DIRECTION('ref_axis',(1.,0.,0.));
#12845=DIRECTION('center_axis',(0.,0.,1.));
#12846=DIRECTION('ref_axis',(1.,0.,0.));
#12847=DIRECTION('center_axis',(0.,0.,1.));
#12848=DIRECTION('ref_axis',(1.,0.,0.));
#12849=DIRECTION('',(0.,0.,1.));
#12850=DIRECTION('center_axis',(0.,0.,-1.));
#12851=DIRECTION('ref_axis',(1.,0.,0.));
#12852=DIRECTION('center_axis',(0.,0.,1.));
#12853=DIRECTION('ref_axis',(1.,0.,0.));
#12854=DIRECTION('center_axis',(0.,0.,1.));
#12855=DIRECTION('ref_axis',(1.,0.,0.));
#12856=DIRECTION('center_axis',(0.,0.,1.));
#12857=DIRECTION('ref_axis',(1.,0.,0.));
#12858=DIRECTION('',(0.,0.,1.));
#12859=DIRECTION('center_axis',(0.,0.,-1.));
#12860=DIRECTION('ref_axis',(1.,0.,0.));
#12861=DIRECTION('center_axis',(0.,0.,1.));
#12862=DIRECTION('ref_axis',(1.,0.,0.));
#12863=DIRECTION('center_axis',(0.,0.,1.));
#12864=DIRECTION('ref_axis',(1.,0.,0.));
#12865=DIRECTION('center_axis',(0.,0.,1.));
#12866=DIRECTION('ref_axis',(1.,0.,0.));
#12867=DIRECTION('',(0.,0.,1.));
#12868=DIRECTION('center_axis',(0.,0.,-1.));
#12869=DIRECTION('ref_axis',(1.,0.,0.));
#12870=DIRECTION('center_axis',(0.,0.,1.));
#12871=DIRECTION('ref_axis',(1.,0.,0.));
#12872=DIRECTION('center_axis',(0.,0.,1.));
#12873=DIRECTION('ref_axis',(1.,0.,0.));
#12874=DIRECTION('',(0.,0.,1.));
#12875=DIRECTION('center_axis',(0.,0.,-1.));
#12876=DIRECTION('ref_axis',(1.,0.,0.));
#12877=DIRECTION('center_axis',(0.,0.,1.));
#12878=DIRECTION('ref_axis',(1.,0.,0.));
#12879=DIRECTION('center_axis',(0.,0.,1.));
#12880=DIRECTION('ref_axis',(1.,0.,0.));
#12881=DIRECTION('',(0.,0.,1.));
#12882=DIRECTION('center_axis',(0.,0.,-1.));
#12883=DIRECTION('ref_axis',(1.,0.,0.));
#12884=DIRECTION('center_axis',(0.,0.,1.));
#12885=DIRECTION('ref_axis',(1.,0.,0.));
#12886=DIRECTION('center_axis',(0.,0.,1.));
#12887=DIRECTION('ref_axis',(1.,0.,0.));
#12888=DIRECTION('',(0.,0.,1.));
#12889=DIRECTION('center_axis',(0.,0.,-1.));
#12890=DIRECTION('ref_axis',(1.,0.,0.));
#12891=DIRECTION('center_axis',(0.,0.,1.));
#12892=DIRECTION('ref_axis',(1.,0.,0.));
#12893=DIRECTION('center_axis',(0.,0.,1.));
#12894=DIRECTION('ref_axis',(1.,0.,0.));
#12895=DIRECTION('',(0.,0.,1.));
#12896=DIRECTION('center_axis',(0.,0.,-1.));
#12897=DIRECTION('ref_axis',(1.,0.,0.));
#12898=DIRECTION('center_axis',(0.,0.,1.));
#12899=DIRECTION('ref_axis',(1.,0.,0.));
#12900=DIRECTION('center_axis',(0.,0.,1.));
#12901=DIRECTION('ref_axis',(1.,0.,0.));
#12902=DIRECTION('center_axis',(0.,0.,1.));
#12903=DIRECTION('ref_axis',(1.,0.,0.));
#12904=DIRECTION('',(0.,0.,1.));
#12905=DIRECTION('center_axis',(0.,0.,-1.));
#12906=DIRECTION('ref_axis',(1.,0.,0.));
#12907=DIRECTION('center_axis',(0.,0.,1.));
#12908=DIRECTION('ref_axis',(1.,0.,0.));
#12909=DIRECTION('center_axis',(0.,0.,1.));
#12910=DIRECTION('ref_axis',(1.,0.,0.));
#12911=DIRECTION('center_axis',(0.,0.,1.));
#12912=DIRECTION('ref_axis',(1.,0.,0.));
#12913=DIRECTION('',(0.,0.,1.));
#12914=DIRECTION('center_axis',(0.,0.,-1.));
#12915=DIRECTION('ref_axis',(1.,0.,0.));
#12916=DIRECTION('center_axis',(0.,0.,1.));
#12917=DIRECTION('ref_axis',(1.,0.,0.));
#12918=DIRECTION('center_axis',(0.,0.,1.));
#12919=DIRECTION('ref_axis',(1.,0.,0.));
#12920=DIRECTION('center_axis',(0.,0.,1.));
#12921=DIRECTION('ref_axis',(1.,0.,0.));
#12922=DIRECTION('',(0.,0.,1.));
#12923=DIRECTION('center_axis',(0.,0.,-1.));
#12924=DIRECTION('ref_axis',(1.,0.,0.));
#12925=DIRECTION('center_axis',(0.,0.,1.));
#12926=DIRECTION('ref_axis',(1.,0.,0.));
#12927=DIRECTION('center_axis',(0.,0.,1.));
#12928=DIRECTION('ref_axis',(1.,0.,0.));
#12929=DIRECTION('center_axis',(0.,0.,1.));
#12930=DIRECTION('ref_axis',(1.,0.,0.));
#12931=DIRECTION('',(0.,0.,1.));
#12932=DIRECTION('center_axis',(0.,0.,-1.));
#12933=DIRECTION('ref_axis',(1.,0.,0.));
#12934=DIRECTION('center_axis',(0.,0.,1.));
#12935=DIRECTION('ref_axis',(1.,0.,0.));
#12936=DIRECTION('center_axis',(0.,0.,1.));
#12937=DIRECTION('ref_axis',(1.,0.,0.));
#12938=DIRECTION('center_axis',(0.,0.,1.));
#12939=DIRECTION('ref_axis',(1.,0.,0.));
#12940=DIRECTION('',(0.,0.,1.));
#12941=DIRECTION('center_axis',(0.,0.,-1.));
#12942=DIRECTION('ref_axis',(1.,0.,0.));
#12943=DIRECTION('center_axis',(0.,0.,1.));
#12944=DIRECTION('ref_axis',(1.,0.,0.));
#12945=DIRECTION('center_axis',(0.,0.,1.));
#12946=DIRECTION('ref_axis',(1.,0.,0.));
#12947=DIRECTION('center_axis',(0.,0.,1.));
#12948=DIRECTION('ref_axis',(1.,0.,0.));
#12949=DIRECTION('',(0.,0.,1.));
#12950=DIRECTION('center_axis',(0.,0.,-1.));
#12951=DIRECTION('ref_axis',(1.,0.,0.));
#12952=DIRECTION('center_axis',(0.,0.,1.));
#12953=DIRECTION('ref_axis',(1.,0.,0.));
#12954=DIRECTION('center_axis',(0.,0.,1.));
#12955=DIRECTION('ref_axis',(1.,0.,0.));
#12956=DIRECTION('center_axis',(0.,0.,1.));
#12957=DIRECTION('ref_axis',(1.,0.,0.));
#12958=DIRECTION('',(0.,0.,1.));
#12959=DIRECTION('center_axis',(0.,0.,-1.));
#12960=DIRECTION('ref_axis',(1.,0.,0.));
#12961=DIRECTION('center_axis',(0.,0.,1.));
#12962=DIRECTION('ref_axis',(1.,0.,0.));
#12963=DIRECTION('center_axis',(0.,1.,0.));
#12964=DIRECTION('ref_axis',(-1.,0.,0.));
#12965=DIRECTION('',(-1.,0.,0.));
#12966=DIRECTION('',(0.,0.,1.));
#12967=DIRECTION('',(-1.,0.,0.));
#12968=DIRECTION('',(0.,0.,1.));
#12969=DIRECTION('center_axis',(1.,0.,0.));
#12970=DIRECTION('ref_axis',(0.,1.,0.));
#12971=DIRECTION('',(0.,1.,0.));
#12972=DIRECTION('',(0.,1.,0.));
#12973=DIRECTION('',(0.,0.,1.));
#12974=DIRECTION('center_axis',(0.,-1.,0.));
#12975=DIRECTION('ref_axis',(1.,0.,0.));
#12976=DIRECTION('',(1.,0.,0.));
#12977=DIRECTION('',(1.,0.,0.));
#12978=DIRECTION('',(0.,0.,1.));
#12979=DIRECTION('center_axis',(-1.,0.,0.));
#12980=DIRECTION('ref_axis',(0.,-1.,0.));
#12981=DIRECTION('',(0.,-1.,0.));
#12982=DIRECTION('',(0.,-1.,0.));
#12983=DIRECTION('center_axis',(0.,0.,1.));
#12984=DIRECTION('ref_axis',(1.,0.,0.));
#12985=DIRECTION('center_axis',(0.,0.,1.));
#12986=DIRECTION('ref_axis',(1.,0.,0.));
#16234=CARTESIAN_POINT('',(0.,0.,0.));
#16235=CARTESIAN_POINT('Origin',(26.2,-2.5,-0.9));
#16236=CARTESIAN_POINT('',(26.035,-2.5,-0.9));
#16237=CARTESIAN_POINT('Origin',(26.2,-2.5,-0.9));
#16238=CARTESIAN_POINT('',(26.035,-2.5,0.));
#16239=CARTESIAN_POINT('',(26.035,-2.5,-0.9));
#16240=CARTESIAN_POINT('Origin',(26.2,-2.5,0.));
#16241=CARTESIAN_POINT('Origin',(26.2,-2.5,-0.9));
#16242=CARTESIAN_POINT('Origin',(26.2,2.5,-0.9));
#16243=CARTESIAN_POINT('',(26.035,2.5,-0.9));
#16244=CARTESIAN_POINT('Origin',(26.2,2.5,-0.9));
#16245=CARTESIAN_POINT('',(26.035,2.5,0.));
#16246=CARTESIAN_POINT('',(26.035,2.5,-0.9));
#16247=CARTESIAN_POINT('Origin',(26.2,2.5,0.));
#16248=CARTESIAN_POINT('Origin',(26.2,2.5,-0.9));
#16249=CARTESIAN_POINT('Origin',(5.8,-2.5,-0.9));
#16250=CARTESIAN_POINT('',(5.635,-2.5,-0.9));
#16251=CARTESIAN_POINT('Origin',(5.8,-2.5,-0.9));
#16252=CARTESIAN_POINT('',(5.635,-2.5,0.));
#16253=CARTESIAN_POINT('',(5.635,-2.5,-0.9));
#16254=CARTESIAN_POINT('Origin',(5.8,-2.5,0.));
#16255=CARTESIAN_POINT('Origin',(5.8,-2.5,-0.9));
#16256=CARTESIAN_POINT('Origin',(5.8,2.5,-0.9));
#16257=CARTESIAN_POINT('',(5.635,2.5,-0.9));
#16258=CARTESIAN_POINT('Origin',(5.8,2.5,-0.9));
#16259=CARTESIAN_POINT('',(5.635,2.5,0.));
#16260=CARTESIAN_POINT('',(5.635,2.5,-0.9));
#16261=CARTESIAN_POINT('Origin',(5.8,2.5,0.));
#16262=CARTESIAN_POINT('Origin',(5.8,2.5,-0.9));
#16263=CARTESIAN_POINT('Origin',(25.,0.,-1.1));
#16264=CARTESIAN_POINT('',(24.835,-2.02066721859312E-17,-1.1));
#16265=CARTESIAN_POINT('Origin',(25.,0.,-1.1));
#16266=CARTESIAN_POINT('',(24.835,2.02066721859312E-17,0.));
#16267=CARTESIAN_POINT('',(24.835,-2.02066721859312E-17,-1.1));
#16268=CARTESIAN_POINT('Origin',(25.,0.,0.));
#16269=CARTESIAN_POINT('Origin',(25.,0.,-1.1));
#16270=CARTESIAN_POINT('Origin',(19.,0.,-1.1));
#16271=CARTESIAN_POINT('',(18.835,-2.02066721859312E-17,-1.1));
#16272=CARTESIAN_POINT('Origin',(19.,0.,-1.1));
#16273=CARTESIAN_POINT('',(18.835,2.02066721859312E-17,0.));
#16274=CARTESIAN_POINT('',(18.835,-2.02066721859312E-17,-1.1));
#16275=CARTESIAN_POINT('Origin',(19.,0.,0.));
#16276=CARTESIAN_POINT('Origin',(19.,0.,-1.1));
#16277=CARTESIAN_POINT('Origin',(13.,0.,-1.1));
#16278=CARTESIAN_POINT('',(12.835,-2.02066721859312E-17,-1.1));
#16279=CARTESIAN_POINT('Origin',(13.,0.,-1.1));
#16280=CARTESIAN_POINT('',(12.835,2.02066721859312E-17,0.));
#16281=CARTESIAN_POINT('',(12.835,-2.02066721859312E-17,-1.1));
#16282=CARTESIAN_POINT('Origin',(13.,0.,0.));
#16283=CARTESIAN_POINT('Origin',(13.,0.,-1.1));
#16284=CARTESIAN_POINT('Origin',(7.,0.,-1.1));
#16285=CARTESIAN_POINT('',(6.835,-2.02066721859313E-17,-1.1));
#16286=CARTESIAN_POINT('Origin',(7.,0.,-1.1));
#16287=CARTESIAN_POINT('',(6.835,2.02066721859313E-17,0.));
#16288=CARTESIAN_POINT('',(6.835,-2.02066721859313E-17,-1.1));
#16289=CARTESIAN_POINT('Origin',(7.,0.,0.));
#16290=CARTESIAN_POINT('Origin',(7.,0.,-1.1));
#16291=CARTESIAN_POINT('Origin',(27.,3.5,-1.3));
#16292=CARTESIAN_POINT('',(26.725,3.5,-1.2));
#16293=CARTESIAN_POINT('Origin',(27.,3.5,-1.2));
#16294=CARTESIAN_POINT('',(26.725,3.5,0.));
#16295=CARTESIAN_POINT('',(26.725,3.5,-1.3));
#16296=CARTESIAN_POINT('Origin',(27.,3.5,0.));
#16297=CARTESIAN_POINT('Origin',(5.,3.5,-1.3));
#16298=CARTESIAN_POINT('',(4.725,3.5,-1.2));
#16299=CARTESIAN_POINT('Origin',(5.,3.5,-1.2));
#16300=CARTESIAN_POINT('',(4.725,3.5,0.));
#16301=CARTESIAN_POINT('',(4.725,3.5,-1.3));
#16302=CARTESIAN_POINT('Origin',(5.,3.5,0.));
#16303=CARTESIAN_POINT('Origin',(27.,-3.5,-1.3));
#16304=CARTESIAN_POINT('',(26.725,-3.5,-1.2));
#16305=CARTESIAN_POINT('Origin',(27.,-3.5,-1.2));
#16306=CARTESIAN_POINT('',(26.725,-3.5,0.));
#16307=CARTESIAN_POINT('',(26.725,-3.5,-1.3));
#16308=CARTESIAN_POINT('Origin',(27.,-3.5,0.));
#16309=CARTESIAN_POINT('Origin',(5.,-3.5,-1.3));
#16310=CARTESIAN_POINT('',(4.725,-3.5,-1.2));
#16311=CARTESIAN_POINT('Origin',(5.,-3.5,-1.2));
#16312=CARTESIAN_POINT('',(4.725,-3.5,0.));
#16313=CARTESIAN_POINT('',(4.725,-3.5,-1.3));
#16314=CARTESIAN_POINT('Origin',(5.,-3.5,0.));
#16315=CARTESIAN_POINT('Origin',(34.8,-1.,-1.1));
#16316=CARTESIAN_POINT('',(34.635,-1.,-1.1));
#16317=CARTESIAN_POINT('Origin',(34.8,-1.,-1.1));
#16318=CARTESIAN_POINT('',(34.635,-1.,0.));
#16319=CARTESIAN_POINT('',(34.635,-1.,-1.1));
#16320=CARTESIAN_POINT('Origin',(34.8,-1.,0.));
#16321=CARTESIAN_POINT('Origin',(34.8,-1.,-1.1));
#16322=CARTESIAN_POINT('Origin',(29.2,1.,-1.1));
#16323=CARTESIAN_POINT('',(29.035,1.,-1.1));
#16324=CARTESIAN_POINT('Origin',(29.2,1.,-1.1));
#16325=CARTESIAN_POINT('',(29.035,1.,0.));
#16326=CARTESIAN_POINT('',(29.035,1.,-1.1));
#16327=CARTESIAN_POINT('Origin',(29.2,1.,0.));
#16328=CARTESIAN_POINT('Origin',(29.2,1.,-1.1));
#16329=CARTESIAN_POINT('Origin',(29.2,-1.,-1.1));
#16330=CARTESIAN_POINT('',(29.035,-1.,-1.1));
#16331=CARTESIAN_POINT('Origin',(29.2,-1.,-1.1));
#16332=CARTESIAN_POINT('',(29.035,-1.,0.));
#16333=CARTESIAN_POINT('',(29.035,-1.,-1.1));
#16334=CARTESIAN_POINT('Origin',(29.2,-1.,0.));
#16335=CARTESIAN_POINT('Origin',(29.2,-1.,-1.1));
#16336=CARTESIAN_POINT('Origin',(34.8,1.,-1.1));
#16337=CARTESIAN_POINT('',(34.635,1.,-1.1));
#16338=CARTESIAN_POINT('Origin',(34.8,1.,-1.1));
#16339=CARTESIAN_POINT('',(34.635,1.,0.));
#16340=CARTESIAN_POINT('',(34.635,1.,-1.1));
#16341=CARTESIAN_POINT('Origin',(34.8,1.,0.));
#16342=CARTESIAN_POINT('Origin',(34.8,1.,-1.1));
#16343=CARTESIAN_POINT('Origin',(2.8,-1.,-1.1));
#16344=CARTESIAN_POINT('',(2.635,-1.,-1.1));
#16345=CARTESIAN_POINT('Origin',(2.8,-1.,-1.1));
#16346=CARTESIAN_POINT('',(2.635,-1.,0.));
#16347=CARTESIAN_POINT('',(2.635,-1.,-1.1));
#16348=CARTESIAN_POINT('Origin',(2.8,-1.,0.));
#16349=CARTESIAN_POINT('Origin',(2.8,-1.,-1.1));
#16350=CARTESIAN_POINT('Origin',(-2.8,1.,-1.1));
#16351=CARTESIAN_POINT('',(-2.965,1.,-1.1));
#16352=CARTESIAN_POINT('Origin',(-2.8,1.,-1.1));
#16353=CARTESIAN_POINT('',(-2.965,1.,0.));
#16354=CARTESIAN_POINT('',(-2.965,1.,-1.1));
#16355=CARTESIAN_POINT('Origin',(-2.8,1.,0.));
#16356=CARTESIAN_POINT('Origin',(-2.8,1.,-1.1));
#16357=CARTESIAN_POINT('Origin',(-2.8,-1.,-1.1));
#16358=CARTESIAN_POINT('',(-2.965,-1.,-1.1));
#16359=CARTESIAN_POINT('Origin',(-2.8,-1.,-1.1));
#16360=CARTESIAN_POINT('',(-2.965,-1.,0.));
#16361=CARTESIAN_POINT('',(-2.965,-1.,-1.1));
#16362=CARTESIAN_POINT('Origin',(-2.8,-1.,0.));
#16363=CARTESIAN_POINT('Origin',(-2.8,-1.,-1.1));
#16364=CARTESIAN_POINT('Origin',(2.8,1.,-1.1));
#16365=CARTESIAN_POINT('',(2.635,1.,-1.1));
#16366=CARTESIAN_POINT('Origin',(2.8,1.,-1.1));
#16367=CARTESIAN_POINT('',(2.635,1.,0.));
#16368=CARTESIAN_POINT('',(2.635,1.,-1.1));
#16369=CARTESIAN_POINT('Origin',(2.8,1.,0.));
#16370=CARTESIAN_POINT('Origin',(2.8,1.,-1.1));
#16371=CARTESIAN_POINT('Origin',(36.,4.5,-1.2));
#16372=CARTESIAN_POINT('',(36.,4.5,-1.2));
#16373=CARTESIAN_POINT('',(-4.,4.5,-1.2));
#16374=CARTESIAN_POINT('',(36.,4.5,-1.2));
#16375=CARTESIAN_POINT('',(-4.,4.5,0.));
#16376=CARTESIAN_POINT('',(-4.,4.5,-1.2));
#16377=CARTESIAN_POINT('',(36.,4.5,0.));
#16378=CARTESIAN_POINT('',(36.,4.5,0.));
#16379=CARTESIAN_POINT('',(36.,4.5,-1.2));
#16380=CARTESIAN_POINT('Origin',(36.,-6.5,-1.2));
#16381=CARTESIAN_POINT('',(36.,-6.5,-1.2));
#16382=CARTESIAN_POINT('',(36.,-6.5,-1.2));
#16383=CARTESIAN_POINT('',(36.,-6.5,0.));
#16384=CARTESIAN_POINT('',(36.,-6.5,0.));
#16385=CARTESIAN_POINT('',(36.,-6.5,-1.2));
#16386=CARTESIAN_POINT('Origin',(-4.,-6.5,-1.2));
#16387=CARTESIAN_POINT('',(-4.,-6.5,-1.2));
#16388=CARTESIAN_POINT('',(-4.,-6.5,-1.2));
#16389=CARTESIAN_POINT('',(-4.,-6.5,0.));
#16390=CARTESIAN_POINT('',(-4.,-6.5,0.));
#16391=CARTESIAN_POINT('',(-4.,-6.5,-1.2));
#16392=CARTESIAN_POINT('Origin',(-4.,4.5,-1.2));
#16393=CARTESIAN_POINT('',(-4.,4.5,-1.2));
#16394=CARTESIAN_POINT('',(-4.,4.5,0.));
#16395=CARTESIAN_POINT('Origin',(16.,-1.,0.));
#16396=CARTESIAN_POINT('Origin',(16.,-1.,-1.2));
#19991=UNCERTAINTY_MEASURE_WITH_UNIT(LENGTH_MEASURE(0.001),#20097,
'DISTANCE_ACCURACY_VALUE',
'Maximum model space distance between geometric entities at asserted c
onnectivities');
#20042=UNCERTAINTY_MEASURE_WITH_UNIT(LENGTH_MEASURE(0.001),#20097,
'DISTANCE_ACCURACY_VALUE',
'Maximum model space distance between geometric entities at asserted c
onnectivities');
#20045=(
GEOMETRIC_REPRESENTATION_CONTEXT(3)
GLOBAL_UNCERTAINTY_ASSIGNED_CONTEXT((#19991))
GLOBAL_UNIT_ASSIGNED_CONTEXT((#20097,#20099,#20100))
REPRESENTATION_CONTEXT('','3D')
);
#20096=(
GEOMETRIC_REPRESENTATION_CONTEXT(3)
GLOBAL_UNCERTAINTY_ASSIGNED_CONTEXT((#20042))
GLOBAL_UNIT_ASSIGNED_CONTEXT((#20097,#20099,#20100))
REPRESENTATION_CONTEXT('','3D')
);
#20097=(
LENGTH_UNIT()
NAMED_UNIT(*)
SI_UNIT(.CENTI.,.METRE.)
);
#20099=(
NAMED_UNIT(*)
PLANE_ANGLE_UNIT()
SI_UNIT($,.RADIAN.)
);
#20100=(
NAMED_UNIT(*)
SI_UNIT($,.STERADIAN.)
SOLID_ANGLE_UNIT()
);
#20103=SHAPE_DEFINITION_REPRESENTATION(#20156,#20314);
#20156=PRODUCT_DEFINITION_SHAPE('',$,#20368);
#20314=SHAPE_REPRESENTATION('',(#11492),#20045);
#20365=PRODUCT_DEFINITION_CONTEXT('part definition',#20526,'design');
#20368=PRODUCT_DEFINITION('Base','Base',#20421,#20365);
#20421=PRODUCT_DEFINITION_FORMATION('',$,#20530);
#20526=APPLICATION_CONTEXT(
'Core Data for Automotive Mechanical Design Process');
#20527=PRODUCT_CONTEXT('part definition',#20526,'mechanical');
#20530=PRODUCT('Base','Base','Base',(#20527));
#20623=COLOUR_RGB('Dark Blue',0.08,0.2,0.34);
#20624=FILL_AREA_STYLE_COLOUR('',#20623);
#20625=FILL_AREA_STYLE('',(#20624));
#20626=SURFACE_STYLE_FILL_AREA(#20625);
#20627=SURFACE_SIDE_STYLE('',(#20626));
#20628=SURFACE_STYLE_USAGE(.BOTH.,#20627);
#20629=PRESENTATION_STYLE_ASSIGNMENT((#20628));
ENDSEC;
END-ISO-10303-21;
